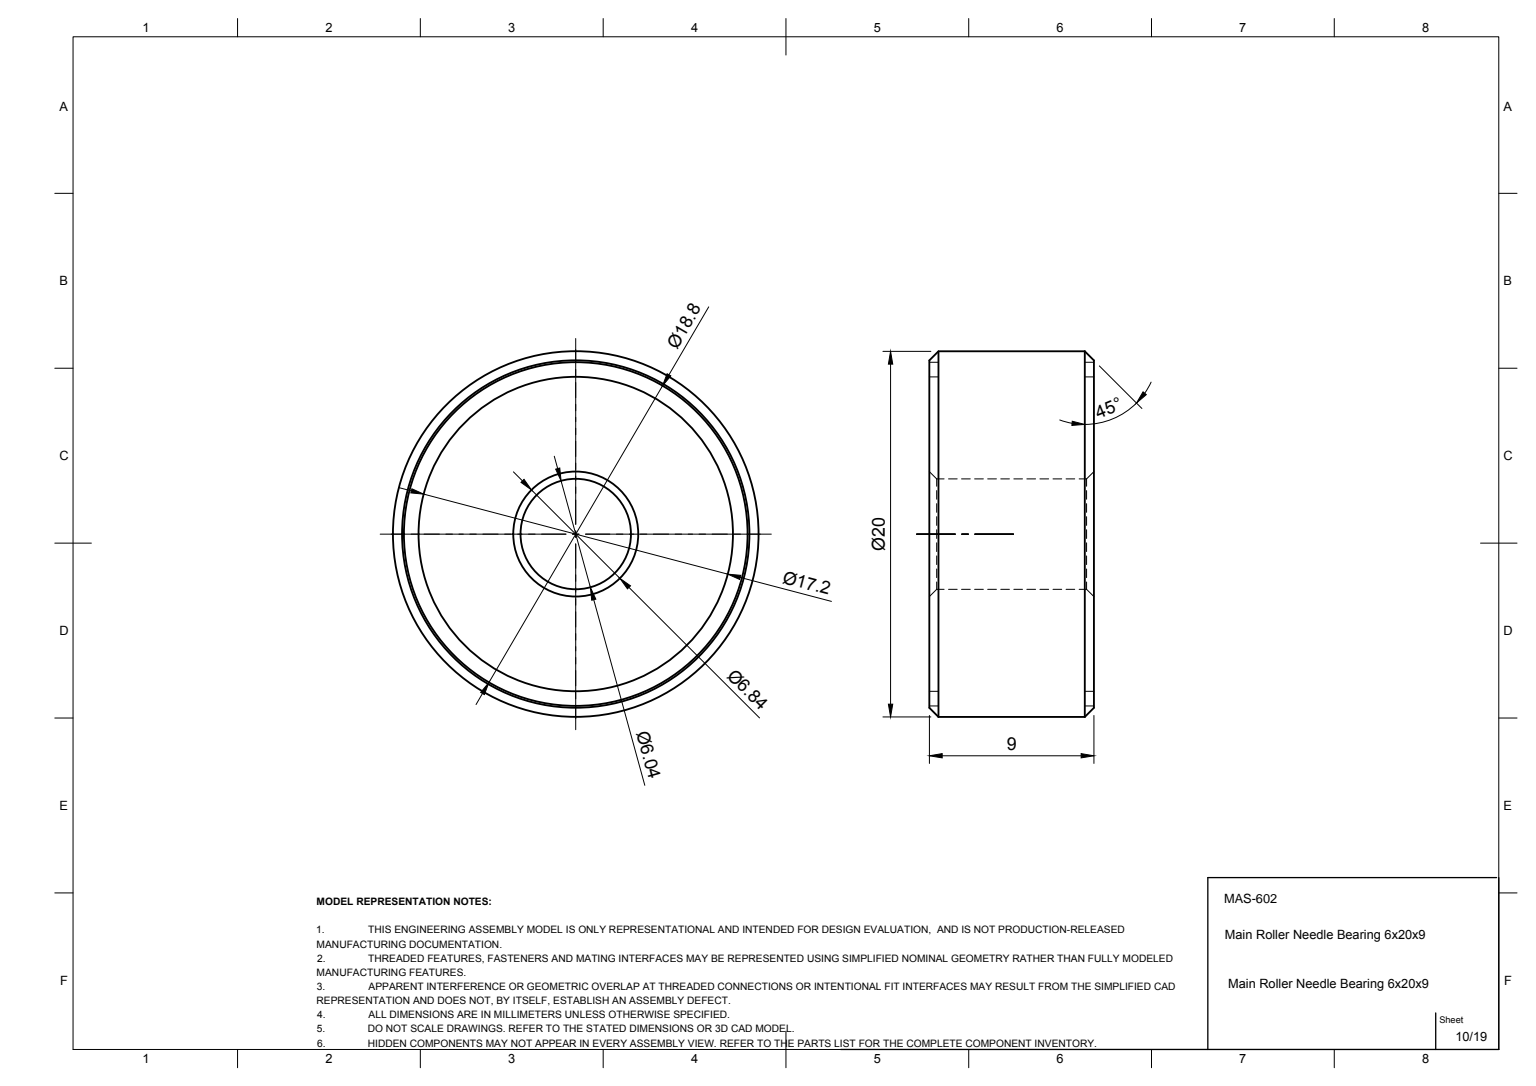
ISO-10303-21;
HEADER;
/* Generated by software containing ST-Developer
 * from STEP Tools, Inc. (www.steptools.com) 
 */

FILE_DESCRIPTION(
/* description */ (''),
/* implementation_level */ '2;1');

FILE_NAME(
/* name */ 'Main Roller Needle Bearing 6x20x9.step',
/* time_stamp */ '2026-10-15T14:42:47-07:00',
/* author */ (''),
/* organization */ (''),
/* preprocessor_version */ 'ST-DEVELOPER v20.2',
/* originating_system */ 'Autodesk Translation Framework v15.15.0.0',
/* authorisation */ '');

FILE_SCHEMA (('AUTOMOTIVE_DESIGN { 1 0 10303 214 3 1 1 }'));
ENDSEC;

DATA;
#10=MECHANICAL_DESIGN_GEOMETRIC_PRESENTATION_REPRESENTATION('',(#244),#85789);
#177=CONICAL_SURFACE('',#10695,0.322,0.785398163397448);
#178=CONICAL_SURFACE('',#10707,0.975,0.785398163397449);
#179=CONICAL_SURFACE('',#10711,0.975,0.785398163397448);
#180=CONICAL_SURFACE('',#10723,0.322,0.785398163397448);
#208=SHAPE_REPRESENTATION_RELATIONSHIP('SRR','None',#85873,#226);
#226=ADVANCED_BREP_SHAPE_REPRESENTATION('',(#262),#85781);
#244=STYLED_ITEM('',(#85972),#262);
#262=MANIFOLD_SOLID_BREP('Body1',#9891);
#461=FACE_BOUND('',#3365,.T.);
#462=FACE_BOUND('',#3368,.T.);
#463=FACE_BOUND('',#3371,.T.);
#464=FACE_BOUND('',#3376,.T.);
#465=FACE_BOUND('',#3379,.T.);
#466=FACE_BOUND('',#3382,.T.);
#1159=PLANE('',#10697);
#1160=PLANE('',#10701);
#1161=PLANE('',#10705);
#1162=PLANE('',#10713);
#1163=PLANE('',#10717);
#1164=PLANE('',#10721);
#1634=LINE('',#77726,#2170);
#1635=LINE('',#77730,#2171);
#1636=LINE('',#77738,#2172);
#1637=LINE('',#77745,#2173);
#1638=LINE('',#77752,#2174);
#1639=LINE('',#77756,#2175);
#1640=LINE('',#77759,#2176);
#1641=LINE('',#77767,#2177);
#1642=LINE('',#77774,#2178);
#1643=LINE('',#77779,#2179);
#2170=VECTOR('',#12586,0.302);
#2171=VECTOR('',#12591,0.322);
#2172=VECTOR('',#12602,0.86);
#2173=VECTOR('',#12611,0.94);
#2174=VECTOR('',#12620,0.975);
#2175=VECTOR('',#12625,1.);
#2176=VECTOR('',#12628,0.975);
#2177=VECTOR('',#12639,0.94);
#2178=VECTOR('',#12648,0.86);
#2179=VECTOR('',#12655,0.322);
#2350=CYLINDRICAL_SURFACE('',#10692,0.302);
#2351=CYLINDRICAL_SURFACE('',#10699,0.86);
#2352=CYLINDRICAL_SURFACE('',#10703,0.94);
#2353=CYLINDRICAL_SURFACE('',#10709,1.);
#2354=CYLINDRICAL_SURFACE('',#10715,0.94);
#2355=CYLINDRICAL_SURFACE('',#10719,0.86);
#2786=FACE_OUTER_BOUND('',#3362,.T.);
#2787=FACE_OUTER_BOUND('',#3363,.T.);
#2788=FACE_OUTER_BOUND('',#3364,.T.);
#2789=FACE_OUTER_BOUND('',#3366,.T.);
#2790=FACE_OUTER_BOUND('',#3367,.T.);
#2791=FACE_OUTER_BOUND('',#3369,.T.);
#2792=FACE_OUTER_BOUND('',#3370,.T.);
#2793=FACE_OUTER_BOUND('',#3372,.T.);
#2794=FACE_OUTER_BOUND('',#3373,.T.);
#2795=FACE_OUTER_BOUND('',#3374,.T.);
#2796=FACE_OUTER_BOUND('',#3375,.T.);
#2797=FACE_OUTER_BOUND('',#3377,.T.);
#2798=FACE_OUTER_BOUND('',#3378,.T.);
#2799=FACE_OUTER_BOUND('',#3380,.T.);
#2800=FACE_OUTER_BOUND('',#3381,.T.);
#2801=FACE_OUTER_BOUND('',#3383,.T.);
#3362=EDGE_LOOP('',(#8757,#8758,#8759,#8760));
#3363=EDGE_LOOP('',(#8761,#8762,#8763,#8764));
#3364=EDGE_LOOP('',(#8765));
#3365=EDGE_LOOP('',(#8766));
#3366=EDGE_LOOP('',(#8767,#8768,#8769,#8770));
#3367=EDGE_LOOP('',(#8771));
#3368=EDGE_LOOP('',(#8772));
#3369=EDGE_LOOP('',(#8773,#8774,#8775,#8776));
#3370=EDGE_LOOP('',(#8777));
#3371=EDGE_LOOP('',(#8778));
#3372=EDGE_LOOP('',(#8779,#8780,#8781,#8782));
#3373=EDGE_LOOP('',(#8783,#8784,#8785,#8786));
#3374=EDGE_LOOP('',(#8787,#8788,#8789,#8790));
#3375=EDGE_LOOP('',(#8791));
#3376=EDGE_LOOP('',(#8792));
#3377=EDGE_LOOP('',(#8793,#8794,#8795,#8796));
#3378=EDGE_LOOP('',(#8797));
#3379=EDGE_LOOP('',(#8798));
#3380=EDGE_LOOP('',(#8799,#8800,#8801,#8802));
#3381=EDGE_LOOP('',(#8803));
#3382=EDGE_LOOP('',(#8804));
#3383=EDGE_LOOP('',(#8805,#8806,#8807,#8808));
#3780=CIRCLE('',#10693,0.302);
#3781=CIRCLE('',#10694,0.302);
#3782=CIRCLE('',#10696,0.342);
#3783=CIRCLE('',#10698,0.86);
#3784=CIRCLE('',#10700,0.86);
#3785=CIRCLE('',#10702,0.94);
#3786=CIRCLE('',#10704,0.94);
#3787=CIRCLE('',#10706,0.95);
#3788=CIRCLE('',#10708,1.);
#3789=CIRCLE('',#10710,1.);
#3790=CIRCLE('',#10712,0.95);
#3791=CIRCLE('',#10714,0.94);
#3792=CIRCLE('',#10716,0.94);
#3793=CIRCLE('',#10718,0.86);
#3794=CIRCLE('',#10720,0.86);
#3795=CIRCLE('',#10722,0.342);
#4717=VERTEX_POINT('',#77723);
#4718=VERTEX_POINT('',#77725);
#4719=VERTEX_POINT('',#77729);
#4720=VERTEX_POINT('',#77733);
#4721=VERTEX_POINT('',#77736);
#4722=VERTEX_POINT('',#77740);
#4723=VERTEX_POINT('',#77743);
#4724=VERTEX_POINT('',#77747);
#4725=VERTEX_POINT('',#77750);
#4726=VERTEX_POINT('',#77754);
#4727=VERTEX_POINT('',#77758);
#4728=VERTEX_POINT('',#77762);
#4729=VERTEX_POINT('',#77765);
#4730=VERTEX_POINT('',#77769);
#4731=VERTEX_POINT('',#77772);
#4732=VERTEX_POINT('',#77776);
#6106=EDGE_CURVE('',#4717,#4717,#3780,.T.);
#6107=EDGE_CURVE('',#4717,#4718,#1634,.T.);
#6108=EDGE_CURVE('',#4718,#4718,#3781,.T.);
#6109=EDGE_CURVE('',#4717,#4719,#1635,.T.);
#6110=EDGE_CURVE('',#4719,#4719,#3782,.T.);
#6111=EDGE_CURVE('',#4720,#4720,#3783,.T.);
#6112=EDGE_CURVE('',#4721,#4721,#3784,.T.);
#6113=EDGE_CURVE('',#4721,#4720,#1636,.T.);
#6114=EDGE_CURVE('',#4722,#4722,#3785,.T.);
#6115=EDGE_CURVE('',#4723,#4723,#3786,.T.);
#6116=EDGE_CURVE('',#4723,#4722,#1637,.T.);
#6117=EDGE_CURVE('',#4724,#4724,#3787,.T.);
#6118=EDGE_CURVE('',#4725,#4725,#3788,.T.);
#6119=EDGE_CURVE('',#4725,#4724,#1638,.T.);
#6120=EDGE_CURVE('',#4726,#4726,#3789,.T.);
#6121=EDGE_CURVE('',#4726,#4725,#1639,.T.);
#6122=EDGE_CURVE('',#4726,#4727,#1640,.T.);
#6123=EDGE_CURVE('',#4727,#4727,#3790,.T.);
#6124=EDGE_CURVE('',#4728,#4728,#3791,.T.);
#6125=EDGE_CURVE('',#4729,#4729,#3792,.T.);
#6126=EDGE_CURVE('',#4729,#4728,#1641,.T.);
#6127=EDGE_CURVE('',#4730,#4730,#3793,.T.);
#6128=EDGE_CURVE('',#4731,#4731,#3794,.T.);
#6129=EDGE_CURVE('',#4731,#4730,#1642,.T.);
#6130=EDGE_CURVE('',#4732,#4732,#3795,.T.);
#6131=EDGE_CURVE('',#4718,#4732,#1643,.T.);
#8757=ORIENTED_EDGE('',*,*,#6106,.F.);
#8758=ORIENTED_EDGE('',*,*,#6107,.T.);
#8759=ORIENTED_EDGE('',*,*,#6108,.T.);
#8760=ORIENTED_EDGE('',*,*,#6107,.F.);
#8761=ORIENTED_EDGE('',*,*,#6106,.T.);
#8762=ORIENTED_EDGE('',*,*,#6109,.T.);
#8763=ORIENTED_EDGE('',*,*,#6110,.F.);
#8764=ORIENTED_EDGE('',*,*,#6109,.F.);
#8765=ORIENTED_EDGE('',*,*,#6111,.F.);
#8766=ORIENTED_EDGE('',*,*,#6110,.T.);
#8767=ORIENTED_EDGE('',*,*,#6112,.F.);
#8768=ORIENTED_EDGE('',*,*,#6113,.T.);
#8769=ORIENTED_EDGE('',*,*,#6111,.T.);
#8770=ORIENTED_EDGE('',*,*,#6113,.F.);
#8771=ORIENTED_EDGE('',*,*,#6114,.F.);
#8772=ORIENTED_EDGE('',*,*,#6112,.T.);
#8773=ORIENTED_EDGE('',*,*,#6115,.F.);
#8774=ORIENTED_EDGE('',*,*,#6116,.T.);
#8775=ORIENTED_EDGE('',*,*,#6114,.T.);
#8776=ORIENTED_EDGE('',*,*,#6116,.F.);
#8777=ORIENTED_EDGE('',*,*,#6117,.F.);
#8778=ORIENTED_EDGE('',*,*,#6115,.T.);
#8779=ORIENTED_EDGE('',*,*,#6118,.F.);
#8780=ORIENTED_EDGE('',*,*,#6119,.T.);
#8781=ORIENTED_EDGE('',*,*,#6117,.T.);
#8782=ORIENTED_EDGE('',*,*,#6119,.F.);
#8783=ORIENTED_EDGE('',*,*,#6120,.F.);
#8784=ORIENTED_EDGE('',*,*,#6121,.T.);
#8785=ORIENTED_EDGE('',*,*,#6118,.T.);
#8786=ORIENTED_EDGE('',*,*,#6121,.F.);
#8787=ORIENTED_EDGE('',*,*,#6120,.T.);
#8788=ORIENTED_EDGE('',*,*,#6122,.T.);
#8789=ORIENTED_EDGE('',*,*,#6123,.F.);
#8790=ORIENTED_EDGE('',*,*,#6122,.F.);
#8791=ORIENTED_EDGE('',*,*,#6123,.T.);
#8792=ORIENTED_EDGE('',*,*,#6124,.F.);
#8793=ORIENTED_EDGE('',*,*,#6125,.F.);
#8794=ORIENTED_EDGE('',*,*,#6126,.T.);
#8795=ORIENTED_EDGE('',*,*,#6124,.T.);
#8796=ORIENTED_EDGE('',*,*,#6126,.F.);
#8797=ORIENTED_EDGE('',*,*,#6125,.T.);
#8798=ORIENTED_EDGE('',*,*,#6127,.F.);
#8799=ORIENTED_EDGE('',*,*,#6128,.F.);
#8800=ORIENTED_EDGE('',*,*,#6129,.T.);
#8801=ORIENTED_EDGE('',*,*,#6127,.T.);
#8802=ORIENTED_EDGE('',*,*,#6129,.F.);
#8803=ORIENTED_EDGE('',*,*,#6128,.T.);
#8804=ORIENTED_EDGE('',*,*,#6130,.F.);
#8805=ORIENTED_EDGE('',*,*,#6108,.F.);
#8806=ORIENTED_EDGE('',*,*,#6131,.T.);
#8807=ORIENTED_EDGE('',*,*,#6130,.T.);
#8808=ORIENTED_EDGE('',*,*,#6131,.F.);
#9764=ADVANCED_FACE('',(#2786),#2350,.F.);
#9765=ADVANCED_FACE('',(#2787),#177,.F.);
#9766=ADVANCED_FACE('',(#2788,#461),#1159,.T.);
#9767=ADVANCED_FACE('',(#2789),#2351,.T.);
#9768=ADVANCED_FACE('',(#2790,#462),#1160,.T.);
#9769=ADVANCED_FACE('',(#2791),#2352,.F.);
#9770=ADVANCED_FACE('',(#2792,#463),#1161,.T.);
#9771=ADVANCED_FACE('',(#2793),#178,.T.);
#9772=ADVANCED_FACE('',(#2794),#2353,.T.);
#9773=ADVANCED_FACE('',(#2795),#179,.T.);
#9774=ADVANCED_FACE('',(#2796,#464),#1162,.T.);
#9775=ADVANCED_FACE('',(#2797),#2354,.F.);
#9776=ADVANCED_FACE('',(#2798,#465),#1163,.T.);
#9777=ADVANCED_FACE('',(#2799),#2355,.T.);
#9778=ADVANCED_FACE('',(#2800,#466),#1164,.T.);
#9779=ADVANCED_FACE('',(#2801),#180,.F.);
#9891=CLOSED_SHELL('',(#9764,#9765,#9766,#9767,#9768,#9769,#9770,#9771,
#9772,#9773,#9774,#9775,#9776,#9777,#9778,#9779));
#10691=AXIS2_PLACEMENT_3D('',#77721,#12580,#12581);
#10692=AXIS2_PLACEMENT_3D('',#77722,#12582,#12583);
#10693=AXIS2_PLACEMENT_3D('',#77724,#12584,#12585);
#10694=AXIS2_PLACEMENT_3D('',#77727,#12587,#12588);
#10695=AXIS2_PLACEMENT_3D('',#77728,#12589,#12590);
#10696=AXIS2_PLACEMENT_3D('',#77731,#12592,#12593);
#10697=AXIS2_PLACEMENT_3D('',#77732,#12594,#12595);
#10698=AXIS2_PLACEMENT_3D('',#77734,#12596,#12597);
#10699=AXIS2_PLACEMENT_3D('',#77735,#12598,#12599);
#10700=AXIS2_PLACEMENT_3D('',#77737,#12600,#12601);
#10701=AXIS2_PLACEMENT_3D('',#77739,#12603,#12604);
#10702=AXIS2_PLACEMENT_3D('',#77741,#12605,#12606);
#10703=AXIS2_PLACEMENT_3D('',#77742,#12607,#12608);
#10704=AXIS2_PLACEMENT_3D('',#77744,#12609,#12610);
#10705=AXIS2_PLACEMENT_3D('',#77746,#12612,#12613);
#10706=AXIS2_PLACEMENT_3D('',#77748,#12614,#12615);
#10707=AXIS2_PLACEMENT_3D('',#77749,#12616,#12617);
#10708=AXIS2_PLACEMENT_3D('',#77751,#12618,#12619);
#10709=AXIS2_PLACEMENT_3D('',#77753,#12621,#12622);
#10710=AXIS2_PLACEMENT_3D('',#77755,#12623,#12624);
#10711=AXIS2_PLACEMENT_3D('',#77757,#12626,#12627);
#10712=AXIS2_PLACEMENT_3D('',#77760,#12629,#12630);
#10713=AXIS2_PLACEMENT_3D('',#77761,#12631,#12632);
#10714=AXIS2_PLACEMENT_3D('',#77763,#12633,#12634);
#10715=AXIS2_PLACEMENT_3D('',#77764,#12635,#12636);
#10716=AXIS2_PLACEMENT_3D('',#77766,#12637,#12638);
#10717=AXIS2_PLACEMENT_3D('',#77768,#12640,#12641);
#10718=AXIS2_PLACEMENT_3D('',#77770,#12642,#12643);
#10719=AXIS2_PLACEMENT_3D('',#77771,#12644,#12645);
#10720=AXIS2_PLACEMENT_3D('',#77773,#12646,#12647);
#10721=AXIS2_PLACEMENT_3D('',#77775,#12649,#12650);
#10722=AXIS2_PLACEMENT_3D('',#77777,#12651,#12652);
#10723=AXIS2_PLACEMENT_3D('',#77778,#12653,#12654);
#12580=DIRECTION('axis',(0.,0.,1.));
#12581=DIRECTION('refdir',(1.,0.,0.));
#12582=DIRECTION('center_axis',(0.,0.,1.));
#12583=DIRECTION('ref_axis',(1.,0.,0.));
#12584=DIRECTION('center_axis',(0.,0.,1.));
#12585=DIRECTION('ref_axis',(1.,0.,0.));
#12586=DIRECTION('',(0.,0.,1.));
#12587=DIRECTION('center_axis',(0.,0.,1.));
#12588=DIRECTION('ref_axis',(1.,0.,0.));
#12589=DIRECTION('center_axis',(0.,0.,-1.));
#12590=DIRECTION('ref_axis',(1.,0.,0.));
#12591=DIRECTION('',(-0.707106781186547,8.65956056235493E-17,-0.707106781186548));
#12592=DIRECTION('center_axis',(0.,0.,1.));
#12593=DIRECTION('ref_axis',(1.,0.,0.));
#12594=DIRECTION('center_axis',(0.,0.,-1.));
#12595=DIRECTION('ref_axis',(-1.,0.,0.));
#12596=DIRECTION('center_axis',(0.,0.,1.));
#12597=DIRECTION('ref_axis',(1.,0.,0.));
#12598=DIRECTION('center_axis',(0.,0.,1.));
#12599=DIRECTION('ref_axis',(1.,0.,0.));
#12600=DIRECTION('center_axis',(0.,0.,1.));
#12601=DIRECTION('ref_axis',(1.,0.,0.));
#12602=DIRECTION('',(0.,0.,-1.));
#12603=DIRECTION('center_axis',(0.,0.,-1.));
#12604=DIRECTION('ref_axis',(-1.,0.,0.));
#12605=DIRECTION('center_axis',(0.,0.,1.));
#12606=DIRECTION('ref_axis',(1.,0.,0.));
#12607=DIRECTION('center_axis',(0.,0.,1.));
#12608=DIRECTION('ref_axis',(1.,0.,0.));
#12609=DIRECTION('center_axis',(0.,0.,1.));
#12610=DIRECTION('ref_axis',(1.,0.,0.));
#12611=DIRECTION('',(0.,0.,1.));
#12612=DIRECTION('center_axis',(0.,0.,-1.));
#12613=DIRECTION('ref_axis',(-1.,0.,0.));
#12614=DIRECTION('center_axis',(0.,0.,1.));
#12615=DIRECTION('ref_axis',(1.,0.,0.));
#12616=DIRECTION('center_axis',(0.,0.,1.));
#12617=DIRECTION('ref_axis',(1.,0.,0.));
#12618=DIRECTION('center_axis',(0.,0.,1.));
#12619=DIRECTION('ref_axis',(1.,0.,0.));
#12620=DIRECTION('',(0.707106781186548,8.65956056235494E-17,-0.707106781186547));
#12621=DIRECTION('center_axis',(0.,0.,1.));
#12622=DIRECTION('ref_axis',(1.,0.,0.));
#12623=DIRECTION('center_axis',(0.,0.,1.));
#12624=DIRECTION('ref_axis',(1.,0.,0.));
#12625=DIRECTION('',(0.,0.,-1.));
#12626=DIRECTION('center_axis',(0.,0.,-1.));
#12627=DIRECTION('ref_axis',(1.,0.,0.));
#12628=DIRECTION('',(0.707106781186547,-8.65956056235493E-17,0.707106781186548));
#12629=DIRECTION('center_axis',(0.,0.,1.));
#12630=DIRECTION('ref_axis',(1.,0.,0.));
#12631=DIRECTION('center_axis',(0.,0.,1.));
#12632=DIRECTION('ref_axis',(1.,0.,0.));
#12633=DIRECTION('center_axis',(0.,0.,1.));
#12634=DIRECTION('ref_axis',(1.,0.,0.));
#12635=DIRECTION('center_axis',(0.,0.,1.));
#12636=DIRECTION('ref_axis',(1.,0.,0.));
#12637=DIRECTION('center_axis',(0.,0.,1.));
#12638=DIRECTION('ref_axis',(1.,0.,0.));
#12639=DIRECTION('',(0.,0.,1.));
#12640=DIRECTION('center_axis',(0.,0.,1.));
#12641=DIRECTION('ref_axis',(1.,0.,0.));
#12642=DIRECTION('center_axis',(0.,0.,1.));
#12643=DIRECTION('ref_axis',(1.,0.,0.));
#12644=DIRECTION('center_axis',(0.,0.,1.));
#12645=DIRECTION('ref_axis',(1.,0.,0.));
#12646=DIRECTION('center_axis',(0.,0.,1.));
#12647=DIRECTION('ref_axis',(1.,0.,0.));
#12648=DIRECTION('',(0.,0.,-1.));
#12649=DIRECTION('center_axis',(0.,0.,1.));
#12650=DIRECTION('ref_axis',(1.,0.,0.));
#12651=DIRECTION('center_axis',(0.,0.,1.));
#12652=DIRECTION('ref_axis',(1.,0.,0.));
#12653=DIRECTION('center_axis',(0.,0.,1.));
#12654=DIRECTION('ref_axis',(1.,0.,0.));
#12655=DIRECTION('',(-0.707106781186547,-8.65956056235493E-17,0.707106781186548));
#77721=CARTESIAN_POINT('',(0.,0.,0.));
#77722=CARTESIAN_POINT('Origin',(0.,0.,0.45));
#77723=CARTESIAN_POINT('',(-0.302,-3.69843333342501E-17,0.04));
#77724=CARTESIAN_POINT('Origin',(0.,0.,0.04));
#77725=CARTESIAN_POINT('',(-0.302,-3.69843333342501E-17,0.86));
#77726=CARTESIAN_POINT('',(-0.302,-3.69843333342501E-17,0.45));
#77727=CARTESIAN_POINT('Origin',(0.,0.,0.86));
#77728=CARTESIAN_POINT('Origin',(0.,0.,0.02));
#77729=CARTESIAN_POINT('',(-0.342,-4.18829205308395E-17,-3.46944695195361E-18));
#77730=CARTESIAN_POINT('',(-0.322,3.94336269325448E-17,0.02));
#77731=CARTESIAN_POINT('Origin',(0.,0.,0.));
#77732=CARTESIAN_POINT('Origin',(0.86,0.,0.));
#77733=CARTESIAN_POINT('',(-0.86,-1.05319624726672E-16,0.));
#77734=CARTESIAN_POINT('Origin',(0.,0.,0.));
#77735=CARTESIAN_POINT('Origin',(0.,0.,0.025));
#77736=CARTESIAN_POINT('',(-0.86,-1.05319624726672E-16,0.05));
#77737=CARTESIAN_POINT('Origin',(0.,0.,0.05));
#77738=CARTESIAN_POINT('',(-0.86,-1.05319624726672E-16,0.025));
#77739=CARTESIAN_POINT('Origin',(0.94,0.,0.05));
#77740=CARTESIAN_POINT('',(-0.94,-1.15116799119851E-16,0.05));
#77741=CARTESIAN_POINT('Origin',(0.,0.,0.05));
#77742=CARTESIAN_POINT('Origin',(0.,0.,0.025));
#77743=CARTESIAN_POINT('',(-0.94,-1.15116799119851E-16,0.));
#77744=CARTESIAN_POINT('Origin',(0.,0.,0.));
#77745=CARTESIAN_POINT('',(-0.94,-1.15116799119851E-16,0.025));
#77746=CARTESIAN_POINT('Origin',(0.95,0.,0.));
#77747=CARTESIAN_POINT('',(-0.95,-1.16341445918999E-16,-6.93889390390723E-18));
#77748=CARTESIAN_POINT('Origin',(0.,0.,0.));
#77749=CARTESIAN_POINT('Origin',(0.,0.,0.025));
#77750=CARTESIAN_POINT('',(-1.,-1.22464679914735E-16,0.05));
#77751=CARTESIAN_POINT('Origin',(0.,0.,0.05));
#77752=CARTESIAN_POINT('',(-0.975,-1.19403062916867E-16,0.025));
#77753=CARTESIAN_POINT('Origin',(0.,0.,0.45));
#77754=CARTESIAN_POINT('',(-1.,-1.22464679914735E-16,0.85));
#77755=CARTESIAN_POINT('Origin',(0.,0.,0.85));
#77756=CARTESIAN_POINT('',(-1.,-1.22464679914735E-16,0.45));
#77757=CARTESIAN_POINT('Origin',(0.,0.,0.875));
#77758=CARTESIAN_POINT('',(-0.95,-1.16341445918999E-16,0.9));
#77759=CARTESIAN_POINT('',(-0.975,1.19403062916867E-16,0.875));
#77760=CARTESIAN_POINT('Origin',(0.,0.,0.9));
#77761=CARTESIAN_POINT('Origin',(0.94,0.,0.9));
#77762=CARTESIAN_POINT('',(-0.94,-1.15116799119851E-16,0.9));
#77763=CARTESIAN_POINT('Origin',(0.,0.,0.9));
#77764=CARTESIAN_POINT('Origin',(0.,0.,0.875));
#77765=CARTESIAN_POINT('',(-0.94,-1.15116799119851E-16,0.85));
#77766=CARTESIAN_POINT('Origin',(0.,0.,0.85));
#77767=CARTESIAN_POINT('',(-0.94,-1.15116799119851E-16,0.875));
#77768=CARTESIAN_POINT('Origin',(0.86,0.,0.85));
#77769=CARTESIAN_POINT('',(-0.86,-1.05319624726672E-16,0.85));
#77770=CARTESIAN_POINT('Origin',(0.,0.,0.85));
#77771=CARTESIAN_POINT('Origin',(0.,0.,0.875));
#77772=CARTESIAN_POINT('',(-0.86,-1.05319624726672E-16,0.9));
#77773=CARTESIAN_POINT('Origin',(0.,0.,0.9));
#77774=CARTESIAN_POINT('',(-0.86,-1.05319624726672E-16,0.875));
#77775=CARTESIAN_POINT('Origin',(0.342,0.,0.9));
#77776=CARTESIAN_POINT('',(-0.342,-4.18829205308395E-17,0.9));
#77777=CARTESIAN_POINT('Origin',(0.,0.,0.9));
#77778=CARTESIAN_POINT('Origin',(0.,0.,0.88));
#77779=CARTESIAN_POINT('',(-0.322,-3.94336269325448E-17,0.88));
#85761=UNCERTAINTY_MEASURE_WITH_UNIT(LENGTH_MEASURE(0.001),#85790,
'DISTANCE_ACCURACY_VALUE',
'Maximum model space distance between geometric entities at asserted c
onnectivities');
#85769=UNCERTAINTY_MEASURE_WITH_UNIT(LENGTH_MEASURE(0.001),#85790,
'DISTANCE_ACCURACY_VALUE',
'Maximum model space distance between geometric entities at asserted c
onnectivities');
#85781=(
GEOMETRIC_REPRESENTATION_CONTEXT(3)
GLOBAL_UNCERTAINTY_ASSIGNED_CONTEXT((#85761))
GLOBAL_UNIT_ASSIGNED_CONTEXT((#85790,#85792,#85793))
REPRESENTATION_CONTEXT('','3D')
);
#85789=(
GEOMETRIC_REPRESENTATION_CONTEXT(3)
GLOBAL_UNCERTAINTY_ASSIGNED_CONTEXT((#85769))
GLOBAL_UNIT_ASSIGNED_CONTEXT((#85790,#85792,#85793))
REPRESENTATION_CONTEXT('','3D')
);
#85790=(
LENGTH_UNIT()
NAMED_UNIT(*)
SI_UNIT(.CENTI.,.METRE.)
);
#85792=(
NAMED_UNIT(*)
PLANE_ANGLE_UNIT()
SI_UNIT($,.RADIAN.)
);
#85793=(
NAMED_UNIT(*)
SI_UNIT($,.STERADIAN.)
SOLID_ANGLE_UNIT()
);
#85805=SHAPE_DEFINITION_REPRESENTATION(#85824,#85873);
#85824=PRODUCT_DEFINITION_SHAPE('',$,#85893);
#85873=SHAPE_REPRESENTATION('',(#10691),#85781);
#85881=PRODUCT_DEFINITION_CONTEXT('part definition',#85940,'design');
#85893=PRODUCT_DEFINITION('Main Roller Needle Bearing 6x20x9',
'Main Roller Needle Bearing 6x20x9',#85912,#85881);
#85912=PRODUCT_DEFINITION_FORMATION('',$,#85953);
#85940=APPLICATION_CONTEXT(
'Core Data for Automotive Mechanical Design Process');
#85941=PRODUCT_CONTEXT('part definition',#85940,'mechanical');
#85953=PRODUCT('Main Roller Needle Bearing 6x20x9',
'Main Roller Needle Bearing 6x20x9',$,(#85941));
#85972=PRESENTATION_STYLE_ASSIGNMENT((#85990));
#85990=SURFACE_STYLE_USAGE(.BOTH.,#86008);
#86008=SURFACE_SIDE_STYLE('',(#86026));
#86026=SURFACE_STYLE_FILL_AREA(#86044);
#86044=FILL_AREA_STYLE('Opaque(206,209,214)',(#86062));
#86062=FILL_AREA_STYLE_COLOUR('Opaque(206,209,214)',#86080);
#86080=COLOUR_RGB('Opaque(206,209,214)', 0.08235294, 0.09019608, 0.10196078);
ENDSEC;
END-ISO-10303-21;
